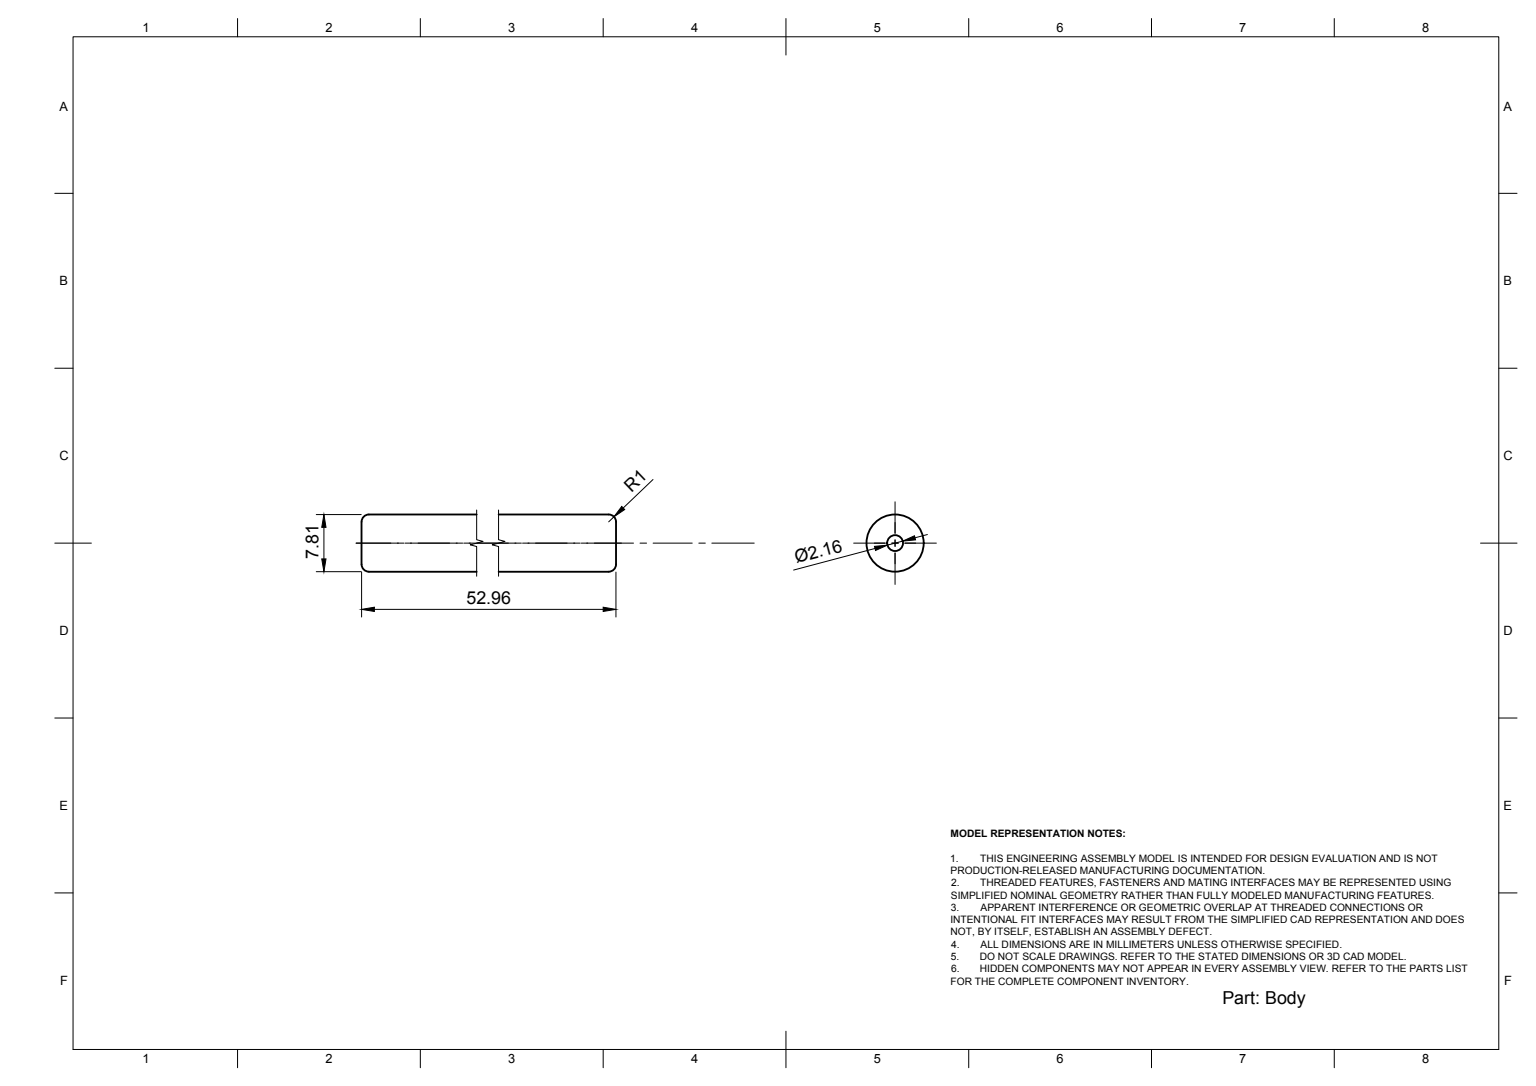
ISO-10303-21;
HEADER;
/* Generated by software containing ST-Developer
 * from STEP Tools, Inc. (www.steptools.com) 
 */

FILE_DESCRIPTION(
/* description */ (''),
/* implementation_level */ '2;1');

FILE_NAME(
/* name */ 'Body.step',
/* time_stamp */ '2026-10-04T22:13:49-07:00',
/* author */ (''),
/* organization */ (''),
/* preprocessor_version */ 'ST-DEVELOPER v20.2',
/* originating_system */ 'Autodesk Translation Framework v15.15.0.0',
/* authorisation */ '');

FILE_SCHEMA (('AUTOMOTIVE_DESIGN { 1 0 10303 214 3 1 1 }'));
ENDSEC;

DATA;
#10=MECHANICAL_DESIGN_GEOMETRIC_PRESENTATION_REPRESENTATION('',(#362),#40734);
#346=SHAPE_REPRESENTATION_RELATIONSHIP('SRR','None',#40767,#354);
#354=ADVANCED_BREP_SHAPE_REPRESENTATION('',(#371),#40727);
#362=STYLED_ITEM('',(#40816),#371);
#371=MANIFOLD_SOLID_BREP('Body1',#3167);
#383=FACE_BOUND('',#599,.T.);
#384=FACE_BOUND('',#604,.T.);
#392=TOROIDAL_SURFACE('',#3290,2.90634189295526,1.);
#393=TOROIDAL_SURFACE('',#3295,2.90634189295527,0.999999999999996);
#398=PLANE('',#3288);
#399=PLANE('',#3298);
#435=FACE_OUTER_BOUND('',#597,.T.);
#436=FACE_OUTER_BOUND('',#598,.T.);
#437=FACE_OUTER_BOUND('',#600,.T.);
#438=FACE_OUTER_BOUND('',#601,.T.);
#439=FACE_OUTER_BOUND('',#602,.T.);
#440=FACE_OUTER_BOUND('',#603,.T.);
#597=EDGE_LOOP('',(#1948,#1949,#1950,#1951));
#598=EDGE_LOOP('',(#1952));
#599=EDGE_LOOP('',(#1953));
#600=EDGE_LOOP('',(#1954,#1955,#1956,#1957));
#601=EDGE_LOOP('',(#1958,#1959,#1960,#1961));
#602=EDGE_LOOP('',(#1962,#1963,#1964,#1965));
#603=EDGE_LOOP('',(#1966));
#604=EDGE_LOOP('',(#1967));
#760=LINE('',#4097,#902);
#761=LINE('',#4109,#903);
#902=VECTOR('',#3531,1.08063175605657);
#903=VECTOR('',#3548,3.90634189295527);
#1051=CIRCLE('',#3286,1.08063175605657);
#1052=CIRCLE('',#3287,1.08063175605657);
#1053=CIRCLE('',#3289,2.90634189295526);
#1054=CIRCLE('',#3291,3.90634189295526);
#1055=CIRCLE('',#3292,1.);
#1056=CIRCLE('',#3294,3.90634189295527);
#1057=CIRCLE('',#3296,2.90634189295526);
#1058=CIRCLE('',#3297,0.999999999999996);
#1099=VERTEX_POINT('',#4094);
#1100=VERTEX_POINT('',#4096);
#1101=VERTEX_POINT('',#4100);
#1102=VERTEX_POINT('',#4103);
#1103=VERTEX_POINT('',#4107);
#1104=VERTEX_POINT('',#4111);
#1450=EDGE_CURVE('',#1099,#1099,#1051,.T.);
#1451=EDGE_CURVE('',#1099,#1100,#760,.T.);
#1452=EDGE_CURVE('',#1100,#1100,#1052,.T.);
#1453=EDGE_CURVE('',#1101,#1101,#1053,.T.);
#1454=EDGE_CURVE('',#1102,#1102,#1054,.T.);
#1455=EDGE_CURVE('',#1102,#1101,#1055,.T.);
#1456=EDGE_CURVE('',#1103,#1103,#1056,.T.);
#1457=EDGE_CURVE('',#1103,#1102,#761,.T.);
#1458=EDGE_CURVE('',#1104,#1104,#1057,.T.);
#1459=EDGE_CURVE('',#1104,#1103,#1058,.T.);
#1948=ORIENTED_EDGE('',*,*,#1450,.F.);
#1949=ORIENTED_EDGE('',*,*,#1451,.T.);
#1950=ORIENTED_EDGE('',*,*,#1452,.F.);
#1951=ORIENTED_EDGE('',*,*,#1451,.F.);
#1952=ORIENTED_EDGE('',*,*,#1453,.F.);
#1953=ORIENTED_EDGE('',*,*,#1452,.T.);
#1954=ORIENTED_EDGE('',*,*,#1454,.F.);
#1955=ORIENTED_EDGE('',*,*,#1455,.T.);
#1956=ORIENTED_EDGE('',*,*,#1453,.T.);
#1957=ORIENTED_EDGE('',*,*,#1455,.F.);
#1958=ORIENTED_EDGE('',*,*,#1456,.F.);
#1959=ORIENTED_EDGE('',*,*,#1457,.T.);
#1960=ORIENTED_EDGE('',*,*,#1454,.T.);
#1961=ORIENTED_EDGE('',*,*,#1457,.F.);
#1962=ORIENTED_EDGE('',*,*,#1458,.F.);
#1963=ORIENTED_EDGE('',*,*,#1459,.T.);
#1964=ORIENTED_EDGE('',*,*,#1456,.T.);
#1965=ORIENTED_EDGE('',*,*,#1459,.F.);
#1966=ORIENTED_EDGE('',*,*,#1458,.T.);
#1967=ORIENTED_EDGE('',*,*,#1450,.T.);
#2895=CYLINDRICAL_SURFACE('',#3285,1.08063175605657);
#2896=CYLINDRICAL_SURFACE('',#3293,3.90634189295527);
#3014=ADVANCED_FACE('',(#435),#2895,.F.);
#3015=ADVANCED_FACE('',(#436,#383),#398,.T.);
#3016=ADVANCED_FACE('',(#437),#392,.T.);
#3017=ADVANCED_FACE('',(#438),#2896,.T.);
#3018=ADVANCED_FACE('',(#439),#393,.T.);
#3019=ADVANCED_FACE('',(#440,#384),#399,.T.);
#3167=CLOSED_SHELL('',(#3014,#3015,#3016,#3017,#3018,#3019));
#3284=AXIS2_PLACEMENT_3D('',#4092,#3525,#3526);
#3285=AXIS2_PLACEMENT_3D('',#4093,#3527,#3528);
#3286=AXIS2_PLACEMENT_3D('',#4095,#3529,#3530);
#3287=AXIS2_PLACEMENT_3D('',#4098,#3532,#3533);
#3288=AXIS2_PLACEMENT_3D('',#4099,#3534,#3535);
#3289=AXIS2_PLACEMENT_3D('',#4101,#3536,#3537);
#3290=AXIS2_PLACEMENT_3D('',#4102,#3538,#3539);
#3291=AXIS2_PLACEMENT_3D('',#4104,#3540,#3541);
#3292=AXIS2_PLACEMENT_3D('',#4105,#3542,#3543);
#3293=AXIS2_PLACEMENT_3D('',#4106,#3544,#3545);
#3294=AXIS2_PLACEMENT_3D('',#4108,#3546,#3547);
#3295=AXIS2_PLACEMENT_3D('',#4110,#3549,#3550);
#3296=AXIS2_PLACEMENT_3D('',#4112,#3551,#3552);
#3297=AXIS2_PLACEMENT_3D('',#4113,#3553,#3554);
#3298=AXIS2_PLACEMENT_3D('',#4114,#3555,#3556);
#3525=DIRECTION('axis',(0.,0.,1.));
#3526=DIRECTION('refdir',(1.,0.,0.));
#3527=DIRECTION('center_axis',(-1.,0.,0.));
#3528=DIRECTION('ref_axis',(0.,1.,0.));
#3529=DIRECTION('center_axis',(-1.,0.,0.));
#3530=DIRECTION('ref_axis',(0.,1.,0.));
#3531=DIRECTION('',(-1.,0.,0.));
#3532=DIRECTION('center_axis',(1.,0.,0.));
#3533=DIRECTION('ref_axis',(0.,1.,0.));
#3534=DIRECTION('center_axis',(-1.,0.,0.));
#3535=DIRECTION('ref_axis',(0.,0.,1.));
#3536=DIRECTION('center_axis',(1.,0.,0.));
#3537=DIRECTION('ref_axis',(0.,0.,-1.));
#3538=DIRECTION('center_axis',(1.,0.,0.));
#3539=DIRECTION('ref_axis',(0.,0.,-1.));
#3540=DIRECTION('center_axis',(1.,0.,0.));
#3541=DIRECTION('ref_axis',(0.,0.,-1.));
#3542=DIRECTION('center_axis',(0.,-1.,-1.22464679914735E-16));
#3543=DIRECTION('ref_axis',(0.,-1.22464679914735E-16,1.));
#3544=DIRECTION('center_axis',(1.,0.,0.));
#3545=DIRECTION('ref_axis',(0.,0.,-1.));
#3546=DIRECTION('center_axis',(1.,0.,0.));
#3547=DIRECTION('ref_axis',(0.,0.,-1.));
#3548=DIRECTION('',(-1.,0.,0.));
#3549=DIRECTION('center_axis',(1.,0.,0.));
#3550=DIRECTION('ref_axis',(0.,0.,-1.));
#3551=DIRECTION('center_axis',(1.,0.,0.));
#3552=DIRECTION('ref_axis',(0.,0.,-1.));
#3553=DIRECTION('center_axis',(0.,-1.,-1.22464679914735E-16));
#3554=DIRECTION('ref_axis',(0.,-1.22464679914735E-16,1.));
#3555=DIRECTION('center_axis',(1.,0.,0.));
#3556=DIRECTION('ref_axis',(0.,0.,-1.));
#4092=CARTESIAN_POINT('',(0.,0.,0.));
#4093=CARTESIAN_POINT('Origin',(67.3063659679149,0.,0.));
#4094=CARTESIAN_POINT('',(67.3063659679149,-1.08063175605657,-1.32339222111166E-16));
#4095=CARTESIAN_POINT('Origin',(67.3063659679149,0.,0.));
#4096=CARTESIAN_POINT('',(14.3512997641764,-1.08063175605657,-1.32339222111166E-16));
#4097=CARTESIAN_POINT('',(67.3063659679149,-1.08063175605657,1.32339222111166E-16));
#4098=CARTESIAN_POINT('Origin',(14.3512997641764,0.,0.));
#4099=CARTESIAN_POINT('Origin',(14.3512997641764,0.,-2.90634189295526));
#4100=CARTESIAN_POINT('',(14.3512997641764,-3.55924229643552E-16,2.90634189295526));
#4101=CARTESIAN_POINT('Origin',(14.3512997641764,0.,0.));
#4102=CARTESIAN_POINT('Origin',(15.3512997641764,0.,0.));
#4103=CARTESIAN_POINT('',(15.3512997641764,-4.78388909558288E-16,3.90634189295526));
#4104=CARTESIAN_POINT('Origin',(15.3512997641764,0.,0.));
#4105=CARTESIAN_POINT('Origin',(15.3512997641764,-3.55924229643552E-16,
2.90634189295526));
#4106=CARTESIAN_POINT('Origin',(40.8288328660457,0.,0.));
#4107=CARTESIAN_POINT('',(66.3063659679149,-4.78388909558288E-16,3.90634189295527));
#4108=CARTESIAN_POINT('Origin',(66.3063659679149,0.,0.));
#4109=CARTESIAN_POINT('',(40.8288328660457,-4.78388909558288E-16,3.90634189295527));
#4110=CARTESIAN_POINT('Origin',(66.3063659679149,0.,0.));
#4111=CARTESIAN_POINT('',(67.3063659679149,-3.55924229643552E-16,2.90634189295526));
#4112=CARTESIAN_POINT('Origin',(67.3063659679149,0.,0.));
#4113=CARTESIAN_POINT('Origin',(66.3063659679149,-3.55924229643553E-16,
2.90634189295527));
#4114=CARTESIAN_POINT('Origin',(67.3063659679149,0.,0.));
#40717=UNCERTAINTY_MEASURE_WITH_UNIT(LENGTH_MEASURE(0.01),#40735,
'DISTANCE_ACCURACY_VALUE',
'Maximum model space distance between geometric entities at asserted c
onnectivities');
#40724=UNCERTAINTY_MEASURE_WITH_UNIT(LENGTH_MEASURE(0.01),#40735,
'DISTANCE_ACCURACY_VALUE',
'Maximum model space distance between geometric entities at asserted c
onnectivities');
#40727=(
GEOMETRIC_REPRESENTATION_CONTEXT(3)
GLOBAL_UNCERTAINTY_ASSIGNED_CONTEXT((#40717))
GLOBAL_UNIT_ASSIGNED_CONTEXT((#40735,#40737,#40738))
REPRESENTATION_CONTEXT('','3D')
);
#40734=(
GEOMETRIC_REPRESENTATION_CONTEXT(3)
GLOBAL_UNCERTAINTY_ASSIGNED_CONTEXT((#40724))
GLOBAL_UNIT_ASSIGNED_CONTEXT((#40735,#40737,#40738))
REPRESENTATION_CONTEXT('','3D')
);
#40735=(
LENGTH_UNIT()
NAMED_UNIT(*)
SI_UNIT(.MILLI.,.METRE.)
);
#40737=(
NAMED_UNIT(*)
PLANE_ANGLE_UNIT()
SI_UNIT($,.RADIAN.)
);
#40738=(
NAMED_UNIT(*)
SI_UNIT($,.STERADIAN.)
SOLID_ANGLE_UNIT()
);
#40741=SHAPE_DEFINITION_REPRESENTATION(#40750,#40767);
#40750=PRODUCT_DEFINITION_SHAPE('',$,#40777);
#40767=SHAPE_REPRESENTATION('',(#3284),#40727);
#40774=PRODUCT_DEFINITION_CONTEXT('part definition',#40803,'design');
#40777=PRODUCT_DEFINITION('Body','Body',#40786,#40774);
#40786=PRODUCT_DEFINITION_FORMATION('',$,#40807);
#40803=APPLICATION_CONTEXT(
'Core Data for Automotive Mechanical Design Process');
#40804=PRODUCT_CONTEXT('part definition',#40803,'mechanical');
#40807=PRODUCT('Body','Body',$,(#40804));
#40816=PRESENTATION_STYLE_ASSIGNMENT((#40819));
#40819=SURFACE_STYLE_USAGE(.BOTH.,#40822);
#40822=SURFACE_SIDE_STYLE('',(#40825));
#40825=SURFACE_STYLE_FILL_AREA(#40828);
#40828=FILL_AREA_STYLE('Opaque(67,67,67)',(#40831));
#40831=FILL_AREA_STYLE_COLOUR('Opaque(67,67,67)',#40834);
#40834=COLOUR_RGB('Opaque(67,67,67)', 0.66274510, 0.83137255, 0.94901961);
ENDSEC;
END-ISO-10303-21;
